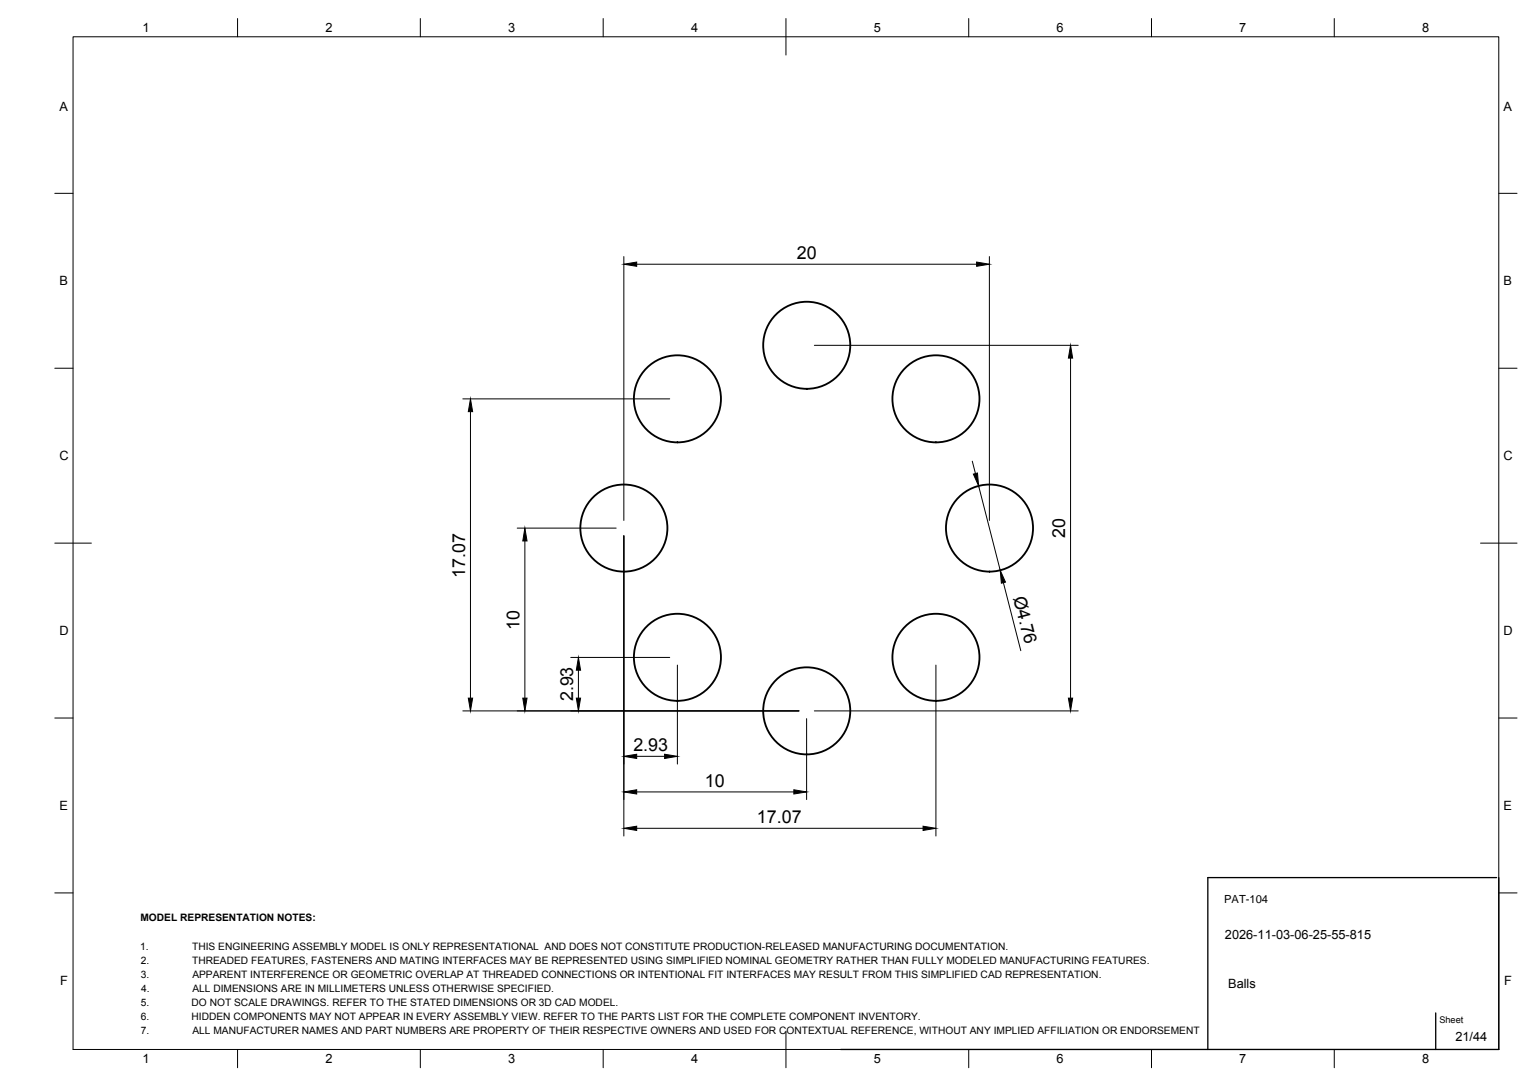
ISO-10303-21;
HEADER;
/* Generated by software containing ST-Developer
 * from STEP Tools, Inc. (www.steptools.com) 
 */

FILE_DESCRIPTION(
/* description */ ('Timing belt drive module 2 mm Pitch Timing 20T-40T'),

/* implementation_level */ '2;1');

FILE_NAME(
/* name */ 'Balls.step',
/* time_stamp */ '2026-10-28T03:25:12-07:00',
/* author */ (''),
/* organization */ (''),
/* preprocessor_version */ 'ST-DEVELOPER v20.2',
/* originating_system */ 'Autodesk Translation Framework v15.17.0.0',
/* authorisation */ '');

FILE_SCHEMA (('AUTOMOTIVE_DESIGN { 1 0 10303 214 3 1 1 }'));
ENDSEC;

DATA;
#10=MECHANICAL_DESIGN_GEOMETRIC_PRESENTATION_REPRESENTATION('',(#542,#543,#544,#545,#546,#547,#548,#549),#17830);
#385=SPHERICAL_SURFACE('',#9918,0.23815);
#386=SPHERICAL_SURFACE('',#9920,0.23815);
#387=SPHERICAL_SURFACE('',#9922,0.23815);
#388=SPHERICAL_SURFACE('',#9924,0.23815);
#389=SPHERICAL_SURFACE('',#9926,0.23815);
#390=SPHERICAL_SURFACE('',#9928,0.23815);
#391=SPHERICAL_SURFACE('',#9930,0.23815);
#392=SPHERICAL_SURFACE('',#9932,0.23815);
#456=SHAPE_REPRESENTATION_RELATIONSHIP('SRR','None',#18027,#499);
#499=ADVANCED_BREP_SHAPE_REPRESENTATION('',(#600,#601,#602,#603,#604,#605,
#606,#607),#17802);
#542=STYLED_ITEM('',(#18317),#600);
#543=STYLED_ITEM('',(#18317),#601);
#544=STYLED_ITEM('',(#18317),#602);
#545=STYLED_ITEM('',(#18317),#603);
#546=STYLED_ITEM('',(#18317),#604);
#547=STYLED_ITEM('',(#18317),#605);
#548=STYLED_ITEM('',(#18317),#606);
#549=STYLED_ITEM('',(#18317),#607);
#600=MANIFOLD_SOLID_BREP('Body1',#8999);
#601=MANIFOLD_SOLID_BREP('Body2',#9000);
#602=MANIFOLD_SOLID_BREP('Body3',#9001);
#603=MANIFOLD_SOLID_BREP('Body4',#9002);
#604=MANIFOLD_SOLID_BREP('Body5',#9003);
#605=MANIFOLD_SOLID_BREP('Body6',#9004);
#606=MANIFOLD_SOLID_BREP('Body7',#9005);
#607=MANIFOLD_SOLID_BREP('Body8',#9006);
#1144=FACE_OUTER_BOUND('',#1741,.T.);
#1145=FACE_OUTER_BOUND('',#1742,.T.);
#1146=FACE_OUTER_BOUND('',#1743,.T.);
#1147=FACE_OUTER_BOUND('',#1744,.T.);
#1148=FACE_OUTER_BOUND('',#1745,.T.);
#1149=FACE_OUTER_BOUND('',#1746,.T.);
#1150=FACE_OUTER_BOUND('',#1747,.T.);
#1151=FACE_OUTER_BOUND('',#1748,.T.);
#1741=EDGE_LOOP('',(#6605,#6606));
#1742=EDGE_LOOP('',(#6607,#6608));
#1743=EDGE_LOOP('',(#6609,#6610));
#1744=EDGE_LOOP('',(#6611,#6612));
#1745=EDGE_LOOP('',(#6613,#6614));
#1746=EDGE_LOOP('',(#6615,#6616));
#1747=EDGE_LOOP('',(#6617,#6618));
#1748=EDGE_LOOP('',(#6619,#6620));
#2338=CIRCLE('',#9919,0.23815);
#2339=CIRCLE('',#9921,0.23815);
#2340=CIRCLE('',#9923,0.23815);
#2341=CIRCLE('',#9925,0.23815);
#2342=CIRCLE('',#9927,0.23815);
#2343=CIRCLE('',#9929,0.23815);
#2344=CIRCLE('',#9931,0.23815);
#2345=CIRCLE('',#9933,0.23815);
#4022=VERTEX_POINT('',#14770);
#4023=VERTEX_POINT('',#14771);
#4024=VERTEX_POINT('',#14774);
#4025=VERTEX_POINT('',#14775);
#4026=VERTEX_POINT('',#14778);
#4027=VERTEX_POINT('',#14779);
#4028=VERTEX_POINT('',#14782);
#4029=VERTEX_POINT('',#14783);
#4030=VERTEX_POINT('',#14786);
#4031=VERTEX_POINT('',#14787);
#4032=VERTEX_POINT('',#14790);
#4033=VERTEX_POINT('',#14791);
#4034=VERTEX_POINT('',#14794);
#4035=VERTEX_POINT('',#14795);
#4036=VERTEX_POINT('',#14798);
#4037=VERTEX_POINT('',#14799);
#4985=EDGE_CURVE('',#4022,#4023,#2338,.T.);
#4986=EDGE_CURVE('',#4024,#4025,#2339,.T.);
#4987=EDGE_CURVE('',#4026,#4027,#2340,.T.);
#4988=EDGE_CURVE('',#4028,#4029,#2341,.T.);
#4989=EDGE_CURVE('',#4030,#4031,#2342,.T.);
#4990=EDGE_CURVE('',#4032,#4033,#2343,.T.);
#4991=EDGE_CURVE('',#4034,#4035,#2344,.T.);
#4992=EDGE_CURVE('',#4036,#4037,#2345,.T.);
#6605=ORIENTED_EDGE('',*,*,#4985,.T.);
#6606=ORIENTED_EDGE('',*,*,#4985,.F.);
#6607=ORIENTED_EDGE('',*,*,#4986,.T.);
#6608=ORIENTED_EDGE('',*,*,#4986,.F.);
#6609=ORIENTED_EDGE('',*,*,#4987,.T.);
#6610=ORIENTED_EDGE('',*,*,#4987,.F.);
#6611=ORIENTED_EDGE('',*,*,#4988,.T.);
#6612=ORIENTED_EDGE('',*,*,#4988,.F.);
#6613=ORIENTED_EDGE('',*,*,#4989,.T.);
#6614=ORIENTED_EDGE('',*,*,#4989,.F.);
#6615=ORIENTED_EDGE('',*,*,#4990,.T.);
#6616=ORIENTED_EDGE('',*,*,#4990,.F.);
#6617=ORIENTED_EDGE('',*,*,#4991,.T.);
#6618=ORIENTED_EDGE('',*,*,#4991,.F.);
#6619=ORIENTED_EDGE('',*,*,#4992,.T.);
#6620=ORIENTED_EDGE('',*,*,#4992,.F.);
#8642=ADVANCED_FACE('',(#1144),#385,.T.);
#8643=ADVANCED_FACE('',(#1145),#386,.T.);
#8644=ADVANCED_FACE('',(#1146),#387,.T.);
#8645=ADVANCED_FACE('',(#1147),#388,.T.);
#8646=ADVANCED_FACE('',(#1148),#389,.T.);
#8647=ADVANCED_FACE('',(#1149),#390,.T.);
#8648=ADVANCED_FACE('',(#1150),#391,.T.);
#8649=ADVANCED_FACE('',(#1151),#392,.T.);
#8999=CLOSED_SHELL('',(#8642));
#9000=CLOSED_SHELL('',(#8643));
#9001=CLOSED_SHELL('',(#8644));
#9002=CLOSED_SHELL('',(#8645));
#9003=CLOSED_SHELL('',(#8646));
#9004=CLOSED_SHELL('',(#8647));
#9005=CLOSED_SHELL('',(#8648));
#9006=CLOSED_SHELL('',(#8649));
#9917=AXIS2_PLACEMENT_3D('',#14768,#11829,#11830);
#9918=AXIS2_PLACEMENT_3D('',#14769,#11831,#11832);
#9919=AXIS2_PLACEMENT_3D('',#14772,#11833,#11834);
#9920=AXIS2_PLACEMENT_3D('',#14773,#11835,#11836);
#9921=AXIS2_PLACEMENT_3D('',#14776,#11837,#11838);
#9922=AXIS2_PLACEMENT_3D('',#14777,#11839,#11840);
#9923=AXIS2_PLACEMENT_3D('',#14780,#11841,#11842);
#9924=AXIS2_PLACEMENT_3D('',#14781,#11843,#11844);
#9925=AXIS2_PLACEMENT_3D('',#14784,#11845,#11846);
#9926=AXIS2_PLACEMENT_3D('',#14785,#11847,#11848);
#9927=AXIS2_PLACEMENT_3D('',#14788,#11849,#11850);
#9928=AXIS2_PLACEMENT_3D('',#14789,#11851,#11852);
#9929=AXIS2_PLACEMENT_3D('',#14792,#11853,#11854);
#9930=AXIS2_PLACEMENT_3D('',#14793,#11855,#11856);
#9931=AXIS2_PLACEMENT_3D('',#14796,#11857,#11858);
#9932=AXIS2_PLACEMENT_3D('',#14797,#11859,#11860);
#9933=AXIS2_PLACEMENT_3D('',#14800,#11861,#11862);
#11829=DIRECTION('axis',(0.,0.,1.));
#11830=DIRECTION('refdir',(1.,0.,0.));
#11831=DIRECTION('center_axis',(0.,0.,1.));
#11832=DIRECTION('ref_axis',(1.,0.,0.));
#11833=DIRECTION('center_axis',(1.22464679914735E-16,-1.,0.));
#11834=DIRECTION('ref_axis',(-1.,-1.22464679914735E-16,0.));
#11835=DIRECTION('center_axis',(0.707106781186548,0.,0.707106781186548));
#11836=DIRECTION('ref_axis',(0.707106781186548,0.,-0.707106781186548));
#11837=DIRECTION('center_axis',(8.65956056235494E-17,-1.,-8.65956056235493E-17));
#11838=DIRECTION('ref_axis',(-0.707106781186547,-1.22464679914735E-16,0.707106781186547));
#11839=DIRECTION('center_axis',(1.,0.,0.));
#11840=DIRECTION('ref_axis',(6.12323399573676E-17,0.,-1.));
#11841=DIRECTION('center_axis',(7.49879891330929E-33,-1.,-1.22464679914735E-16));
#11842=DIRECTION('ref_axis',(-6.12323399573676E-17,-1.22464679914735E-16,
1.));
#11843=DIRECTION('center_axis',(0.707106781186548,0.,-0.707106781186548));
#11844=DIRECTION('ref_axis',(-0.707106781186548,0.,-0.707106781186548));
#11845=DIRECTION('center_axis',(-8.65956056235493E-17,-1.,-8.65956056235494E-17));
#11846=DIRECTION('ref_axis',(0.707106781186547,-1.22464679914735E-16,0.707106781186547));
#11847=DIRECTION('center_axis',(0.,0.,-1.));
#11848=DIRECTION('ref_axis',(-1.,0.,-1.22464679914735E-16));
#11849=DIRECTION('center_axis',(-1.22464679914735E-16,-1.,-1.49975978266186E-32));
#11850=DIRECTION('ref_axis',(1.,-1.22464679914735E-16,1.22464679914735E-16));
#11851=DIRECTION('center_axis',(-0.707106781186547,0.,-0.707106781186548));
#11852=DIRECTION('ref_axis',(-0.707106781186548,0.,0.707106781186547));
#11853=DIRECTION('center_axis',(-8.65956056235493E-17,-1.,8.65956056235493E-17));
#11854=DIRECTION('ref_axis',(0.707106781186548,-1.22464679914735E-16,-0.707106781186547));
#11855=DIRECTION('center_axis',(-1.,0.,0.));
#11856=DIRECTION('ref_axis',(-1.83697019872103E-16,0.,1.));
#11857=DIRECTION('center_axis',(-2.24963967399279E-32,-1.,1.22464679914735E-16));
#11858=DIRECTION('ref_axis',(1.83697019872103E-16,-1.22464679914735E-16,
-1.));
#11859=DIRECTION('center_axis',(-0.707106781186548,0.,0.707106781186548));
#11860=DIRECTION('ref_axis',(0.707106781186547,0.,0.707106781186548));
#11861=DIRECTION('center_axis',(8.65956056235493E-17,-1.,8.65956056235493E-17));
#11862=DIRECTION('ref_axis',(-0.707106781186547,-1.22464679914735E-16,-0.707106781186548));
#14768=CARTESIAN_POINT('',(0.,0.,0.));
#14769=CARTESIAN_POINT('Origin',(1.,0.,0.));
#14770=CARTESIAN_POINT('',(1.,-1.78583896120461E-33,0.23815));
#14771=CARTESIAN_POINT('',(1.,-1.78583896120461E-33,-0.23815));
#14772=CARTESIAN_POINT('Origin',(1.,0.,0.));
#14773=CARTESIAN_POINT('Origin',(0.707106781186548,0.,-0.707106781186547));
#14774=CARTESIAN_POINT('',(0.875504261126124,-1.78583896120461E-33,-0.538709301246971));
#14775=CARTESIAN_POINT('',(0.538709301246971,-1.78583896120461E-33,-0.875504261126124));
#14776=CARTESIAN_POINT('Origin',(0.707106781186548,0.,-0.707106781186547));
#14777=CARTESIAN_POINT('Origin',(6.12323399573677E-17,0.,-1.));
#14778=CARTESIAN_POINT('',(0.23815,-1.78583896120461E-33,-1.));
#14779=CARTESIAN_POINT('',(-0.23815,-1.78583896120461E-33,-1.));
#14780=CARTESIAN_POINT('Origin',(6.12323399573677E-17,0.,-1.));
#14781=CARTESIAN_POINT('Origin',(-0.707106781186547,0.,-0.707106781186548));
#14782=CARTESIAN_POINT('',(-0.538709301246971,-1.78583896120461E-33,-0.875504261126124));
#14783=CARTESIAN_POINT('',(-0.875504261126124,-1.78583896120461E-33,-0.538709301246971));
#14784=CARTESIAN_POINT('Origin',(-0.707106781186547,0.,-0.707106781186548));
#14785=CARTESIAN_POINT('Origin',(-1.,0.,-1.22464679914735E-16));
#14786=CARTESIAN_POINT('',(-1.,-1.78583896120461E-33,-0.23815));
#14787=CARTESIAN_POINT('',(-1.,-1.78583896120461E-33,0.23815));
#14788=CARTESIAN_POINT('Origin',(-1.,0.,-1.22464679914735E-16));
#14789=CARTESIAN_POINT('Origin',(-0.707106781186548,0.,0.707106781186547));
#14790=CARTESIAN_POINT('',(-0.875504261126124,-7.94881478324376E-33,0.538709301246971));
#14791=CARTESIAN_POINT('',(-0.538709301246971,4.37713686083455E-33,0.875504261126124));
#14792=CARTESIAN_POINT('Origin',(-0.707106781186548,0.,0.707106781186547));
#14793=CARTESIAN_POINT('Origin',(-1.83697019872103E-16,0.,1.));
#14794=CARTESIAN_POINT('',(-0.23815,-1.78583896120461E-33,1.));
#14795=CARTESIAN_POINT('',(0.23815,-1.78583896120461E-33,1.));
#14796=CARTESIAN_POINT('Origin',(-1.83697019872103E-16,0.,1.));
#14797=CARTESIAN_POINT('Origin',(0.707106781186547,0.,0.707106781186548));
#14798=CARTESIAN_POINT('',(0.538709301246971,-4.86732687222419E-33,0.875504261126124));
#14799=CARTESIAN_POINT('',(0.875504261126124,1.29564894981497E-33,0.538709301246971));
#14800=CARTESIAN_POINT('Origin',(0.707106781186547,0.,0.707106781186548));
#17752=UNCERTAINTY_MEASURE_WITH_UNIT(LENGTH_MEASURE(0.001),#17831,
'DISTANCE_ACCURACY_VALUE',
'Maximum model space distance between geometric entities at asserted c
onnectivities');
#17780=UNCERTAINTY_MEASURE_WITH_UNIT(LENGTH_MEASURE(0.001),#17831,
'DISTANCE_ACCURACY_VALUE',
'Maximum model space distance between geometric entities at asserted c
onnectivities');
#17802=(
GEOMETRIC_REPRESENTATION_CONTEXT(3)
GLOBAL_UNCERTAINTY_ASSIGNED_CONTEXT((#17752))
GLOBAL_UNIT_ASSIGNED_CONTEXT((#17831,#17833,#17834))
REPRESENTATION_CONTEXT('','3D')
);
#17830=(
GEOMETRIC_REPRESENTATION_CONTEXT(3)
GLOBAL_UNCERTAINTY_ASSIGNED_CONTEXT((#17780))
GLOBAL_UNIT_ASSIGNED_CONTEXT((#17831,#17833,#17834))
REPRESENTATION_CONTEXT('','3D')
);
#17831=(
LENGTH_UNIT()
NAMED_UNIT(*)
SI_UNIT(.CENTI.,.METRE.)
);
#17833=(
NAMED_UNIT(*)
PLANE_ANGLE_UNIT()
SI_UNIT($,.RADIAN.)
);
#17834=(
NAMED_UNIT(*)
SI_UNIT($,.STERADIAN.)
SOLID_ANGLE_UNIT()
);
#17856=SHAPE_DEFINITION_REPRESENTATION(#17905,#18027);
#17905=PRODUCT_DEFINITION_SHAPE('',$,#18077);
#18027=SHAPE_REPRESENTATION('',(#9917),#17802);
#18055=PRODUCT_DEFINITION_CONTEXT('part definition',#18204,'design');
#18077=PRODUCT_DEFINITION('Balls','Balls',#18126,#18055);
#18126=PRODUCT_DEFINITION_FORMATION('',$,#18227);
#18204=APPLICATION_CONTEXT(
'Core Data for Automotive Mechanical Design Process');
#18205=PRODUCT_CONTEXT('part definition',#18204,'mechanical');
#18227=PRODUCT('Balls','Balls','Balls',(#18205));
#18311=COLOUR_RGB('Grey',0.48,0.52,0.57);
#18312=FILL_AREA_STYLE_COLOUR('',#18311);
#18313=FILL_AREA_STYLE('',(#18312));
#18314=SURFACE_STYLE_FILL_AREA(#18313);
#18315=SURFACE_SIDE_STYLE('',(#18314));
#18316=SURFACE_STYLE_USAGE(.BOTH.,#18315);
#18317=PRESENTATION_STYLE_ASSIGNMENT((#18316));
ENDSEC;
END-ISO-10303-21;
